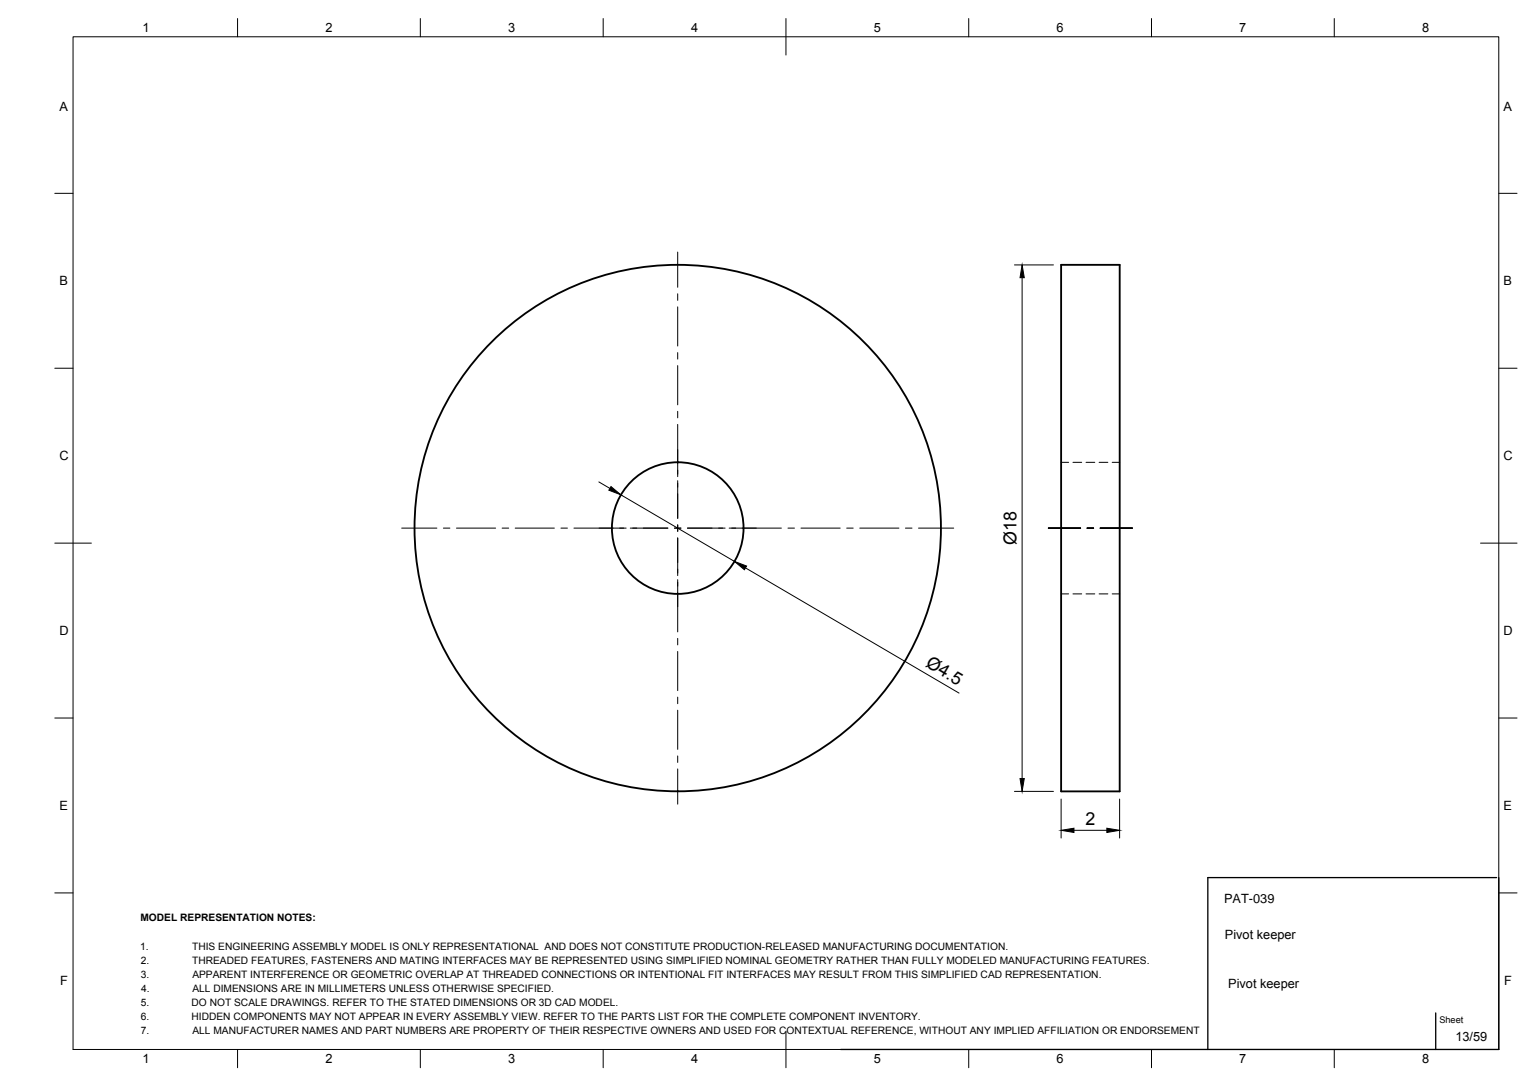
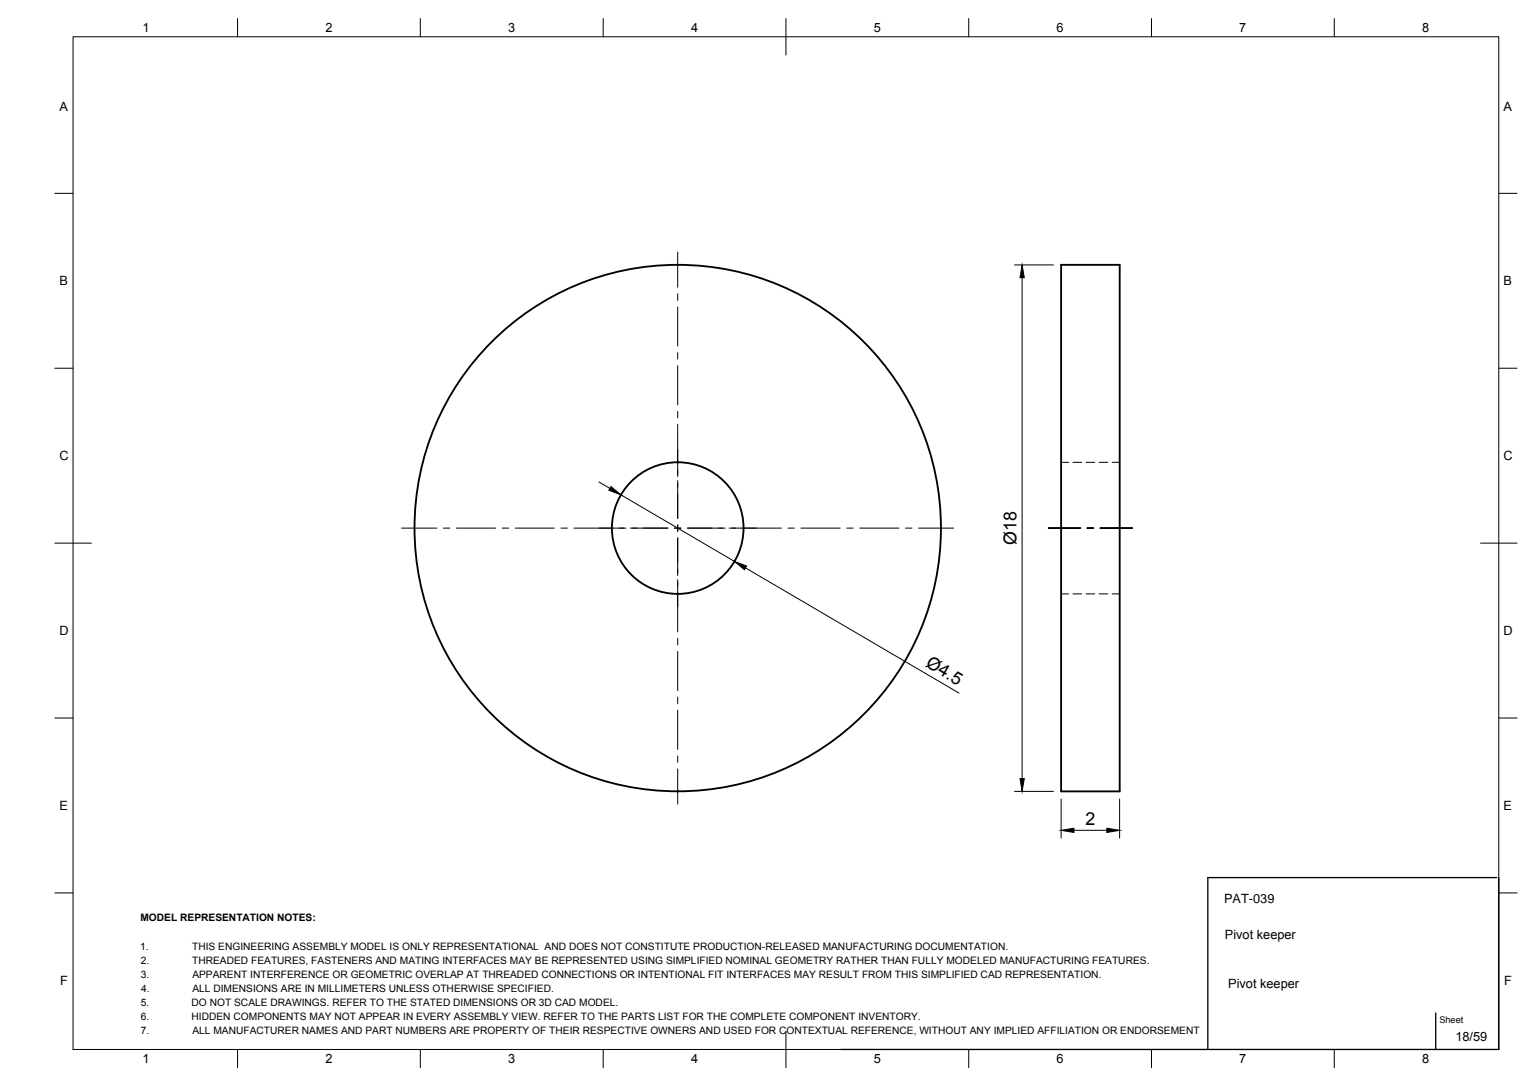
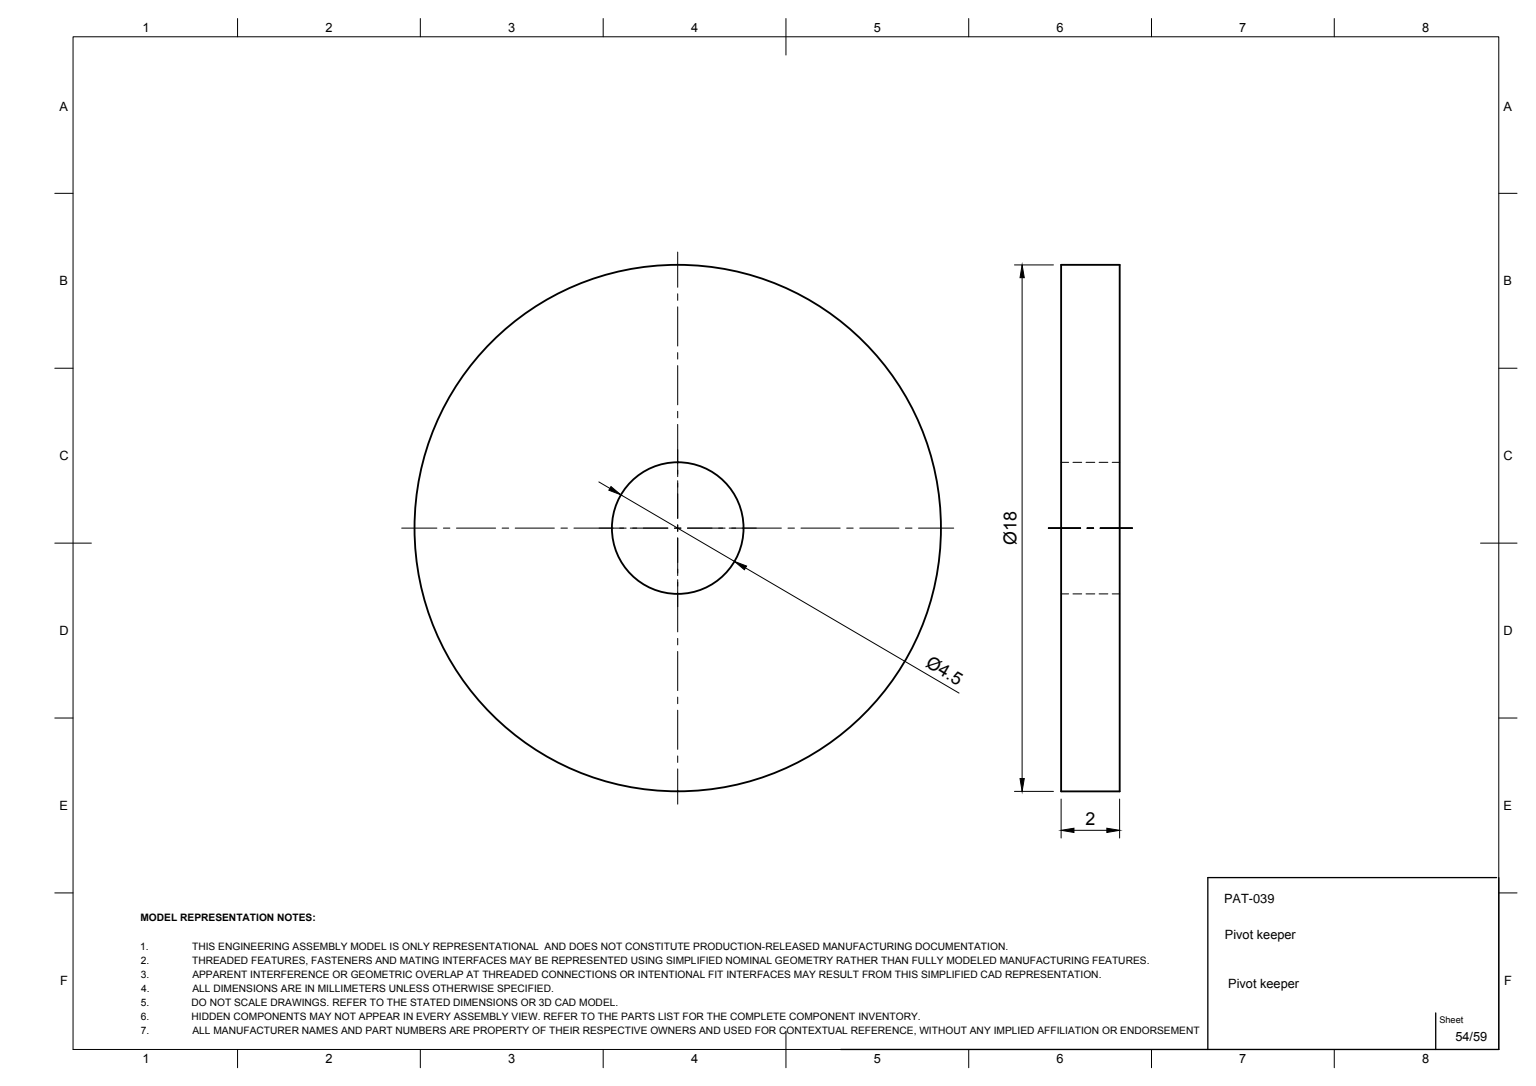
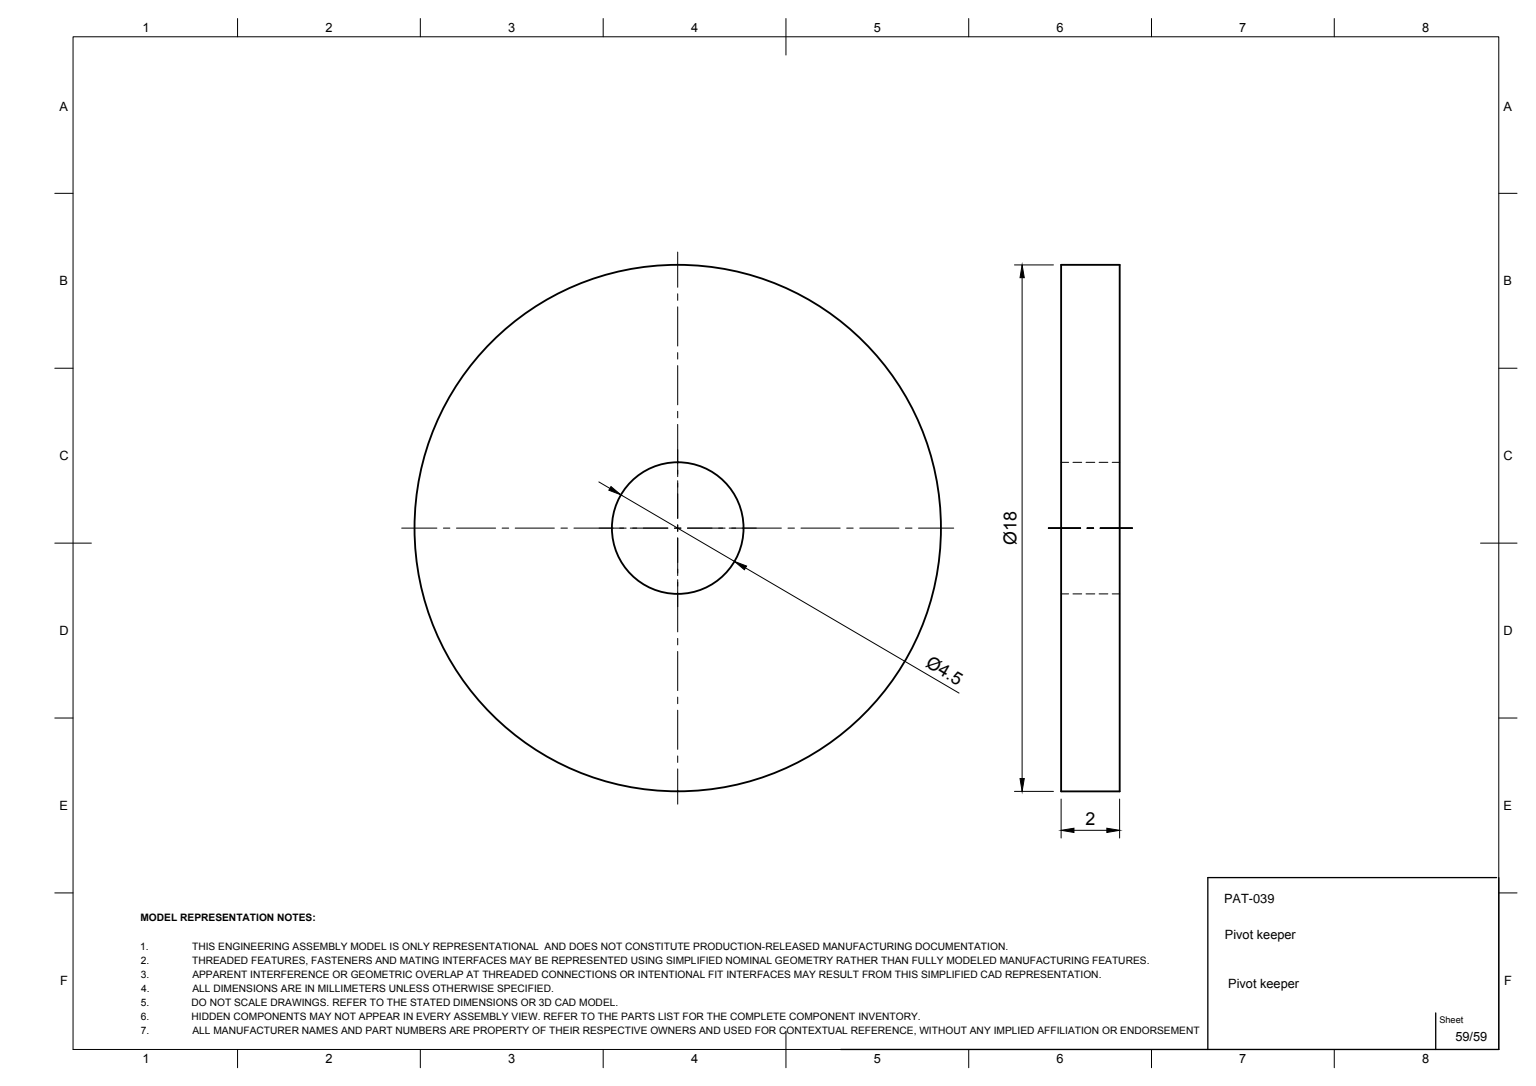
ISO-10303-21;
HEADER;
/* Generated by software containing ST-Developer
 * from STEP Tools, Inc. (www.steptools.com) 
 */

FILE_DESCRIPTION(
/* description */ ('Four-bar parallelogram arm'),
/* implementation_level */ '2;1');

FILE_NAME(
/* name */ 'Pivot keeper.step',
/* time_stamp */ '2026-10-28T03:24:55-07:00',
/* author */ (''),
/* organization */ (''),
/* preprocessor_version */ 'ST-DEVELOPER v20.2',
/* originating_system */ 'Autodesk Translation Framework v15.17.0.0',
/* authorisation */ '');

FILE_SCHEMA (('AUTOMOTIVE_DESIGN { 1 0 10303 214 3 1 1 }'));
ENDSEC;

DATA;
#10=MECHANICAL_DESIGN_GEOMETRIC_PRESENTATION_REPRESENTATION('',(#630),#14512);
#530=SHAPE_REPRESENTATION_RELATIONSHIP('SRR','None',#14751,#580);
#580=ADVANCED_BREP_SHAPE_REPRESENTATION('',(#688),#14466);
#630=STYLED_ITEM('',(#15101),#688);
#688=MANIFOLD_SOLID_BREP('Body1',#7334);
#783=FACE_BOUND('',#1742,.T.);
#784=FACE_BOUND('',#1744,.T.);
#1046=PLANE('',#8085);
#1047=PLANE('',#8086);
#1271=FACE_OUTER_BOUND('',#1739,.T.);
#1272=FACE_OUTER_BOUND('',#1740,.T.);
#1273=FACE_OUTER_BOUND('',#1741,.T.);
#1274=FACE_OUTER_BOUND('',#1743,.T.);
#1739=EDGE_LOOP('',(#5288,#5289,#5290,#5291));
#1740=EDGE_LOOP('',(#5292,#5293,#5294,#5295));
#1741=EDGE_LOOP('',(#5296));
#1742=EDGE_LOOP('',(#5297));
#1743=EDGE_LOOP('',(#5298));
#1744=EDGE_LOOP('',(#5299));
#2402=LINE('',#11763,#2796);
#2403=LINE('',#11769,#2797);
#2796=VECTOR('',#9346,0.225);
#2797=VECTOR('',#9353,0.9);
#3160=CIRCLE('',#8080,0.225);
#3161=CIRCLE('',#8081,0.225);
#3162=CIRCLE('',#8083,0.9);
#3163=CIRCLE('',#8084,0.9);
#3645=VERTEX_POINT('',#11760);
#3646=VERTEX_POINT('',#11762);
#3647=VERTEX_POINT('',#11766);
#3648=VERTEX_POINT('',#11768);
#4275=EDGE_CURVE('',#3645,#3645,#3160,.T.);
#4276=EDGE_CURVE('',#3645,#3646,#2402,.T.);
#4277=EDGE_CURVE('',#3646,#3646,#3161,.T.);
#4278=EDGE_CURVE('',#3647,#3647,#3162,.T.);
#4279=EDGE_CURVE('',#3647,#3648,#2403,.T.);
#4280=EDGE_CURVE('',#3648,#3648,#3163,.T.);
#5288=ORIENTED_EDGE('',*,*,#4275,.F.);
#5289=ORIENTED_EDGE('',*,*,#4276,.T.);
#5290=ORIENTED_EDGE('',*,*,#4277,.T.);
#5291=ORIENTED_EDGE('',*,*,#4276,.F.);
#5292=ORIENTED_EDGE('',*,*,#4278,.F.);
#5293=ORIENTED_EDGE('',*,*,#4279,.T.);
#5294=ORIENTED_EDGE('',*,*,#4280,.T.);
#5295=ORIENTED_EDGE('',*,*,#4279,.F.);
#5296=ORIENTED_EDGE('',*,*,#4278,.T.);
#5297=ORIENTED_EDGE('',*,*,#4275,.T.);
#5298=ORIENTED_EDGE('',*,*,#4280,.F.);
#5299=ORIENTED_EDGE('',*,*,#4277,.F.);
#6744=CYLINDRICAL_SURFACE('',#8079,0.225);
#6745=CYLINDRICAL_SURFACE('',#8082,0.9);
#6976=ADVANCED_FACE('',(#1271),#6744,.F.);
#6977=ADVANCED_FACE('',(#1272),#6745,.T.);
#6978=ADVANCED_FACE('',(#1273,#783),#1046,.T.);
#6979=ADVANCED_FACE('',(#1274,#784),#1047,.F.);
#7334=CLOSED_SHELL('',(#6976,#6977,#6978,#6979));
#8078=AXIS2_PLACEMENT_3D('',#11758,#9340,#9341);
#8079=AXIS2_PLACEMENT_3D('',#11759,#9342,#9343);
#8080=AXIS2_PLACEMENT_3D('',#11761,#9344,#9345);
#8081=AXIS2_PLACEMENT_3D('',#11764,#9347,#9348);
#8082=AXIS2_PLACEMENT_3D('',#11765,#9349,#9350);
#8083=AXIS2_PLACEMENT_3D('',#11767,#9351,#9352);
#8084=AXIS2_PLACEMENT_3D('',#11770,#9354,#9355);
#8085=AXIS2_PLACEMENT_3D('',#11771,#9356,#9357);
#8086=AXIS2_PLACEMENT_3D('',#11772,#9358,#9359);
#9340=DIRECTION('axis',(0.,0.,1.));
#9341=DIRECTION('refdir',(1.,0.,0.));
#9342=DIRECTION('center_axis',(0.,1.,0.));
#9343=DIRECTION('ref_axis',(1.,0.,0.));
#9344=DIRECTION('center_axis',(0.,-1.,0.));
#9345=DIRECTION('ref_axis',(1.,0.,0.));
#9346=DIRECTION('',(0.,-1.,0.));
#9347=DIRECTION('center_axis',(0.,-1.,0.));
#9348=DIRECTION('ref_axis',(1.,0.,0.));
#9349=DIRECTION('center_axis',(0.,1.,0.));
#9350=DIRECTION('ref_axis',(1.,0.,0.));
#9351=DIRECTION('center_axis',(0.,1.,0.));
#9352=DIRECTION('ref_axis',(1.,0.,0.));
#9353=DIRECTION('',(0.,-1.,0.));
#9354=DIRECTION('center_axis',(0.,1.,0.));
#9355=DIRECTION('ref_axis',(1.,0.,0.));
#9356=DIRECTION('center_axis',(0.,1.,0.));
#9357=DIRECTION('ref_axis',(1.,0.,0.));
#9358=DIRECTION('center_axis',(0.,1.,0.));
#9359=DIRECTION('ref_axis',(1.,0.,0.));
#11758=CARTESIAN_POINT('',(0.,0.,0.));
#11759=CARTESIAN_POINT('Origin',(0.,-4.2,8.));
#11760=CARTESIAN_POINT('',(-0.225,-4.,8.));
#11761=CARTESIAN_POINT('Origin',(0.,-4.,8.));
#11762=CARTESIAN_POINT('',(-0.225,-4.2,8.));
#11763=CARTESIAN_POINT('',(-0.225,-4.2,8.));
#11764=CARTESIAN_POINT('Origin',(0.,-4.2,8.));
#11765=CARTESIAN_POINT('Origin',(0.,-4.2,8.));
#11766=CARTESIAN_POINT('',(-0.9,-4.,8.));
#11767=CARTESIAN_POINT('Origin',(0.,-4.,8.));
#11768=CARTESIAN_POINT('',(-0.9,-4.2,8.));
#11769=CARTESIAN_POINT('',(-0.9,-4.2,8.));
#11770=CARTESIAN_POINT('Origin',(0.,-4.2,8.));
#11771=CARTESIAN_POINT('Origin',(0.,-4.,8.));
#11772=CARTESIAN_POINT('Origin',(0.,-4.2,8.));
#14409=UNCERTAINTY_MEASURE_WITH_UNIT(LENGTH_MEASURE(0.001),#14513,
'DISTANCE_ACCURACY_VALUE',
'Maximum model space distance between geometric entities at asserted c
onnectivities');
#14455=UNCERTAINTY_MEASURE_WITH_UNIT(LENGTH_MEASURE(0.001),#14513,
'DISTANCE_ACCURACY_VALUE',
'Maximum model space distance between geometric entities at asserted c
onnectivities');
#14466=(
GEOMETRIC_REPRESENTATION_CONTEXT(3)
GLOBAL_UNCERTAINTY_ASSIGNED_CONTEXT((#14409))
GLOBAL_UNIT_ASSIGNED_CONTEXT((#14513,#14515,#14516))
REPRESENTATION_CONTEXT('','3D')
);
#14512=(
GEOMETRIC_REPRESENTATION_CONTEXT(3)
GLOBAL_UNCERTAINTY_ASSIGNED_CONTEXT((#14455))
GLOBAL_UNIT_ASSIGNED_CONTEXT((#14513,#14515,#14516))
REPRESENTATION_CONTEXT('','3D')
);
#14513=(
LENGTH_UNIT()
NAMED_UNIT(*)
SI_UNIT(.CENTI.,.METRE.)
);
#14515=(
NAMED_UNIT(*)
PLANE_ANGLE_UNIT()
SI_UNIT($,.RADIAN.)
);
#14516=(
NAMED_UNIT(*)
SI_UNIT($,.STERADIAN.)
SOLID_ANGLE_UNIT()
);
#14527=SHAPE_DEFINITION_REPRESENTATION(#14583,#14751);
#14583=PRODUCT_DEFINITION_SHAPE('',$,#14808);
#14751=SHAPE_REPRESENTATION('',(#8078),#14466);
#14797=PRODUCT_DEFINITION_CONTEXT('part definition',#14967,'design');
#14808=PRODUCT_DEFINITION('Pivot keeper','Pivot keeper',#14864,#14797);
#14864=PRODUCT_DEFINITION_FORMATION('',$,#14979);
#14967=APPLICATION_CONTEXT(
'Core Data for Automotive Mechanical Design Process');
#14968=PRODUCT_CONTEXT('part definition',#14967,'mechanical');
#14979=PRODUCT('Pivot keeper','Pivot keeper','Pivot keeper',(#14968));
#15095=COLOUR_RGB('Off White',0.89,0.88,0.83);
#15096=FILL_AREA_STYLE_COLOUR('',#15095);
#15097=FILL_AREA_STYLE('',(#15096));
#15098=SURFACE_STYLE_FILL_AREA(#15097);
#15099=SURFACE_SIDE_STYLE('',(#15098));
#15100=SURFACE_STYLE_USAGE(.BOTH.,#15099);
#15101=PRESENTATION_STYLE_ASSIGNMENT((#15100));
ENDSEC;
END-ISO-10303-21;
